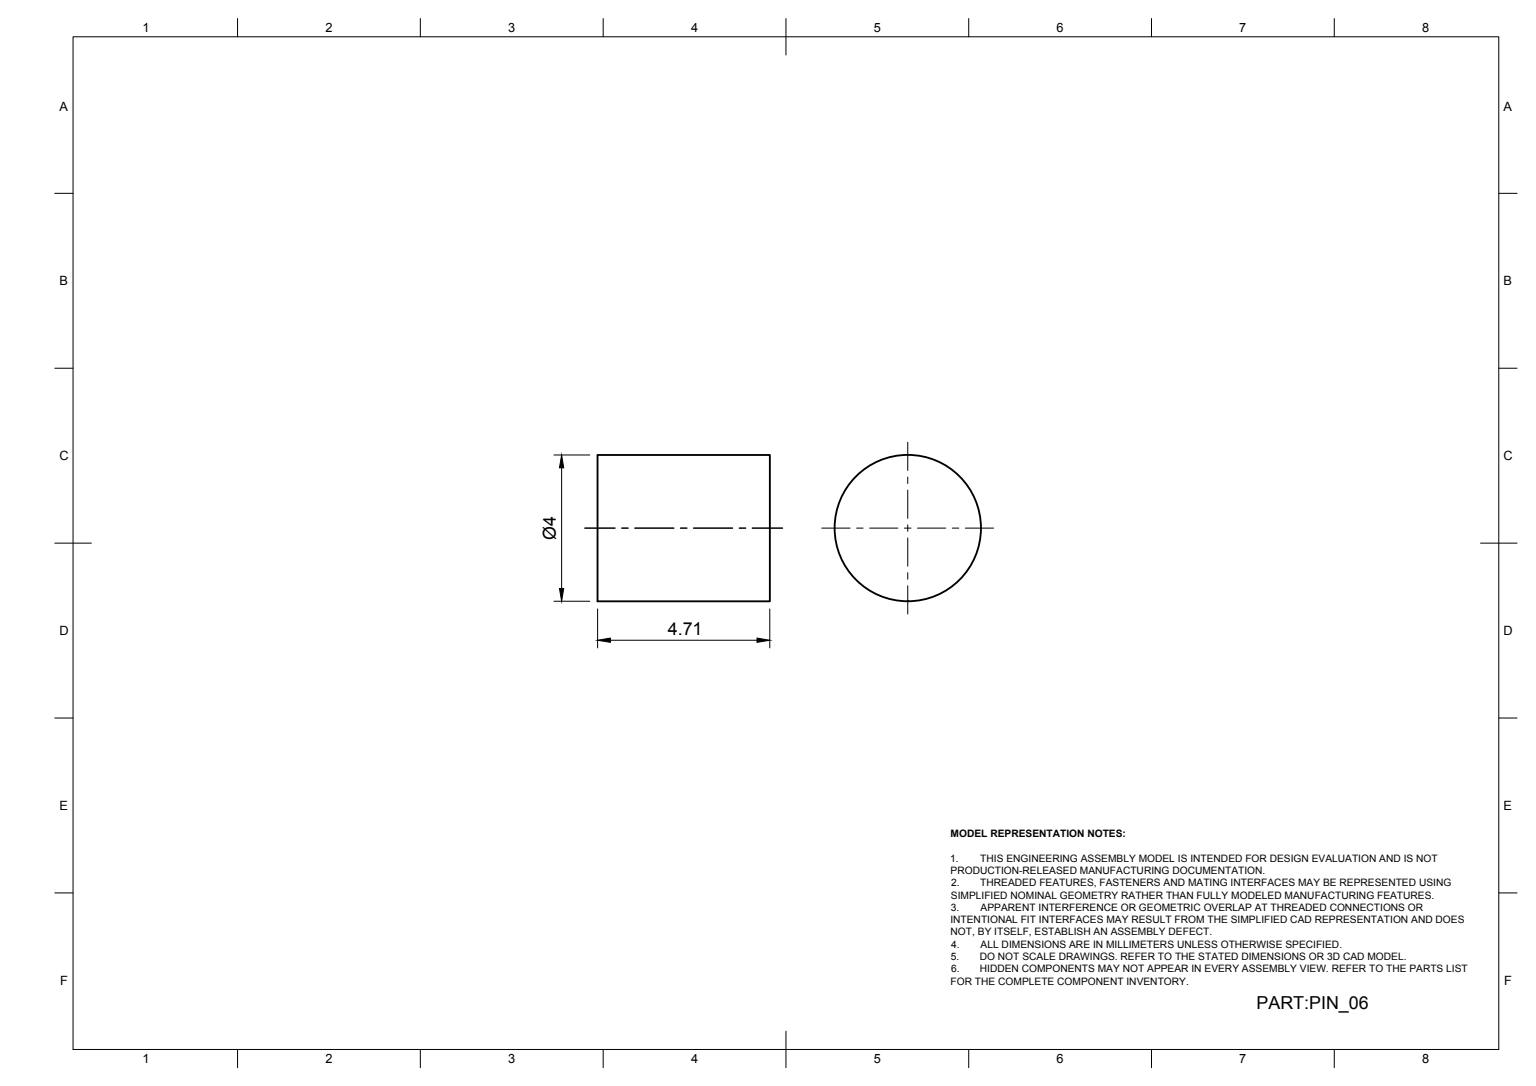
ISO-10303-21;
HEADER;
/* Generated by software containing ST-Developer
 * from STEP Tools, Inc. (www.steptools.com) 
 */

FILE_DESCRIPTION(
/* description */ (''),
/* implementation_level */ '2;1');

FILE_NAME(
/* name */ 'Pin_06.step',
/* time_stamp */ '2026-10-05T13:12:53-07:00',
/* author */ (''),
/* organization */ (''),
/* preprocessor_version */ 'ST-DEVELOPER v20.2',
/* originating_system */ 'Autodesk Translation Framework v15.15.0.0',
/* authorisation */ '');

FILE_SCHEMA (('AUTOMOTIVE_DESIGN { 1 0 10303 214 3 1 1 }'));
ENDSEC;

DATA;
#10=MECHANICAL_DESIGN_GEOMETRIC_PRESENTATION_REPRESENTATION('',(#66),#5912);
#50=SHAPE_REPRESENTATION_RELATIONSHIP('SRR','None',#5951,#58);
#58=ADVANCED_BREP_SHAPE_REPRESENTATION('',(#74),#5911);
#66=STYLED_ITEM('',(#5994),#74);
#74=MANIFOLD_SOLID_BREP('Body1',#3477);
#167=CYLINDRICAL_SURFACE('',#3873,2.);
#347=FACE_OUTER_BOUND('',#550,.T.);
#348=FACE_OUTER_BOUND('',#551,.T.);
#349=FACE_OUTER_BOUND('',#552,.T.);
#550=EDGE_LOOP('',(#3154,#3155,#3156,#3157));
#551=EDGE_LOOP('',(#3158));
#552=EDGE_LOOP('',(#3159));
#653=CIRCLE('',#3874,2.);
#654=CIRCLE('',#3875,2.);
#1019=LINE('',#5881,#1384);
#1384=VECTOR('',#4866,2.);
#1703=VERTEX_POINT('',#5878);
#1704=VERTEX_POINT('',#5880);
#2187=EDGE_CURVE('',#1703,#1703,#653,.T.);
#2188=EDGE_CURVE('',#1703,#1704,#1019,.T.);
#2189=EDGE_CURVE('',#1704,#1704,#654,.T.);
#3154=ORIENTED_EDGE('',*,*,#2187,.T.);
#3155=ORIENTED_EDGE('',*,*,#2188,.T.);
#3156=ORIENTED_EDGE('',*,*,#2189,.T.);
#3157=ORIENTED_EDGE('',*,*,#2188,.F.);
#3158=ORIENTED_EDGE('',*,*,#2187,.F.);
#3159=ORIENTED_EDGE('',*,*,#2189,.F.);
#3286=PLANE('',#3876);
#3287=PLANE('',#3877);
#3467=ADVANCED_FACE('',(#347),#167,.T.);
#3468=ADVANCED_FACE('',(#348),#3286,.F.);
#3469=ADVANCED_FACE('',(#349),#3287,.T.);
#3477=CLOSED_SHELL('',(#3467,#3468,#3469));
#3872=AXIS2_PLACEMENT_3D('',#5876,#4860,#4861);
#3873=AXIS2_PLACEMENT_3D('',#5877,#4862,#4863);
#3874=AXIS2_PLACEMENT_3D('',#5879,#4864,#4865);
#3875=AXIS2_PLACEMENT_3D('',#5882,#4867,#4868);
#3876=AXIS2_PLACEMENT_3D('',#5883,#4869,#4870);
#3877=AXIS2_PLACEMENT_3D('',#5884,#4871,#4872);
#4860=DIRECTION('axis',(0.,0.,1.));
#4861=DIRECTION('refdir',(1.,0.,0.));
#4862=DIRECTION('center_axis',(2.44876222201709E-16,-0.0208291764396898,
-0.999783049170591));
#4863=DIRECTION('ref_axis',(1.,-7.39048179408127E-33,2.44929359829471E-16));
#4864=DIRECTION('center_axis',(-2.44876222201709E-16,0.0208291764396898,
0.999783049170591));
#4865=DIRECTION('ref_axis',(1.,-7.39048179408127E-33,2.44929359829471E-16));
#4866=DIRECTION('',(-2.44876222201709E-16,0.0208291764396898,0.999783049170591));
#4867=DIRECTION('center_axis',(2.44876222201709E-16,-0.0208291764396898,
-0.999783049170591));
#4868=DIRECTION('ref_axis',(1.,-7.39048179408127E-33,2.44929359829471E-16));
#4869=DIRECTION('center_axis',(-2.44876222201709E-16,0.0208291764396898,
0.999783049170591));
#4870=DIRECTION('ref_axis',(1.,-7.39048179408127E-33,2.44929359829471E-16));
#4871=DIRECTION('center_axis',(-2.44876222201709E-16,0.0208291764396898,
0.999783049170591));
#4872=DIRECTION('ref_axis',(1.,-7.39048179408127E-33,2.44929359829471E-16));
#5876=CARTESIAN_POINT('',(0.,0.,0.));
#5877=CARTESIAN_POINT('Origin',(55.4902124404907,-4.00000013411045,0.145828066207017));
#5878=CARTESIAN_POINT('',(53.4902124404907,-4.00000013411045,0.145828066207017));
#5879=CARTESIAN_POINT('Origin',(55.4902124404907,-4.00000013411045,0.145828066207017));
#5880=CARTESIAN_POINT('',(53.4902124404907,-3.90187388390307,4.85580601084967));
#5881=CARTESIAN_POINT('',(53.4902124404907,-4.00000013411045,0.145828066207016));
#5882=CARTESIAN_POINT('Origin',(55.4902124404907,-3.90187388390307,4.85580601084967));
#5883=CARTESIAN_POINT('Origin',(55.4902124404907,-4.00000013411045,0.145828066207017));
#5884=CARTESIAN_POINT('Origin',(55.4902124404907,-3.90187388390307,4.85580601084967));
#5901=UNCERTAINTY_MEASURE_WITH_UNIT(LENGTH_MEASURE(0.01),#5913,
'DISTANCE_ACCURACY_VALUE',
'Maximum model space distance between geometric entities at asserted c
onnectivities');
#5902=UNCERTAINTY_MEASURE_WITH_UNIT(LENGTH_MEASURE(0.01),#5913,
'DISTANCE_ACCURACY_VALUE',
'Maximum model space distance between geometric entities at asserted c
onnectivities');
#5911=(
GEOMETRIC_REPRESENTATION_CONTEXT(3)
GLOBAL_UNCERTAINTY_ASSIGNED_CONTEXT((#5901))
GLOBAL_UNIT_ASSIGNED_CONTEXT((#5913,#5915,#5916))
REPRESENTATION_CONTEXT('','3D')
);
#5912=(
GEOMETRIC_REPRESENTATION_CONTEXT(3)
GLOBAL_UNCERTAINTY_ASSIGNED_CONTEXT((#5902))
GLOBAL_UNIT_ASSIGNED_CONTEXT((#5913,#5915,#5916))
REPRESENTATION_CONTEXT('','3D')
);
#5913=(
LENGTH_UNIT()
NAMED_UNIT(*)
SI_UNIT(.MILLI.,.METRE.)
);
#5915=(
NAMED_UNIT(*)
PLANE_ANGLE_UNIT()
SI_UNIT($,.RADIAN.)
);
#5916=(
NAMED_UNIT(*)
SI_UNIT($,.STERADIAN.)
SOLID_ANGLE_UNIT()
);
#5925=SHAPE_DEFINITION_REPRESENTATION(#5934,#5951);
#5934=PRODUCT_DEFINITION_SHAPE('',$,#5961);
#5951=SHAPE_REPRESENTATION('',(#3872),#5911);
#5952=PRODUCT_DEFINITION_CONTEXT('part definition',#5981,'design');
#5961=PRODUCT_DEFINITION('Pin_06','Pin_06',#5970,#5952);
#5970=PRODUCT_DEFINITION_FORMATION('',$,#5991);
#5981=APPLICATION_CONTEXT(
'Core Data for Automotive Mechanical Design Process');
#5982=PRODUCT_CONTEXT('part definition',#5981,'mechanical');
#5991=PRODUCT('Pin_06','Pin_06',$,(#5982));
#5994=PRESENTATION_STYLE_ASSIGNMENT((#5997));
#5997=SURFACE_STYLE_USAGE(.BOTH.,#6000);
#6000=SURFACE_SIDE_STYLE('',(#6003));
#6003=SURFACE_STYLE_FILL_AREA(#6006);
#6006=FILL_AREA_STYLE('Opaque(160,160,160)',(#6009));
#6009=FILL_AREA_STYLE_COLOUR('Opaque(160,160,160)',#6012);
#6012=COLOUR_RGB('Opaque(160,160,160)', 0.31764706, 0.68627451, 0.89019608);
ENDSEC;
END-ISO-10303-21;
